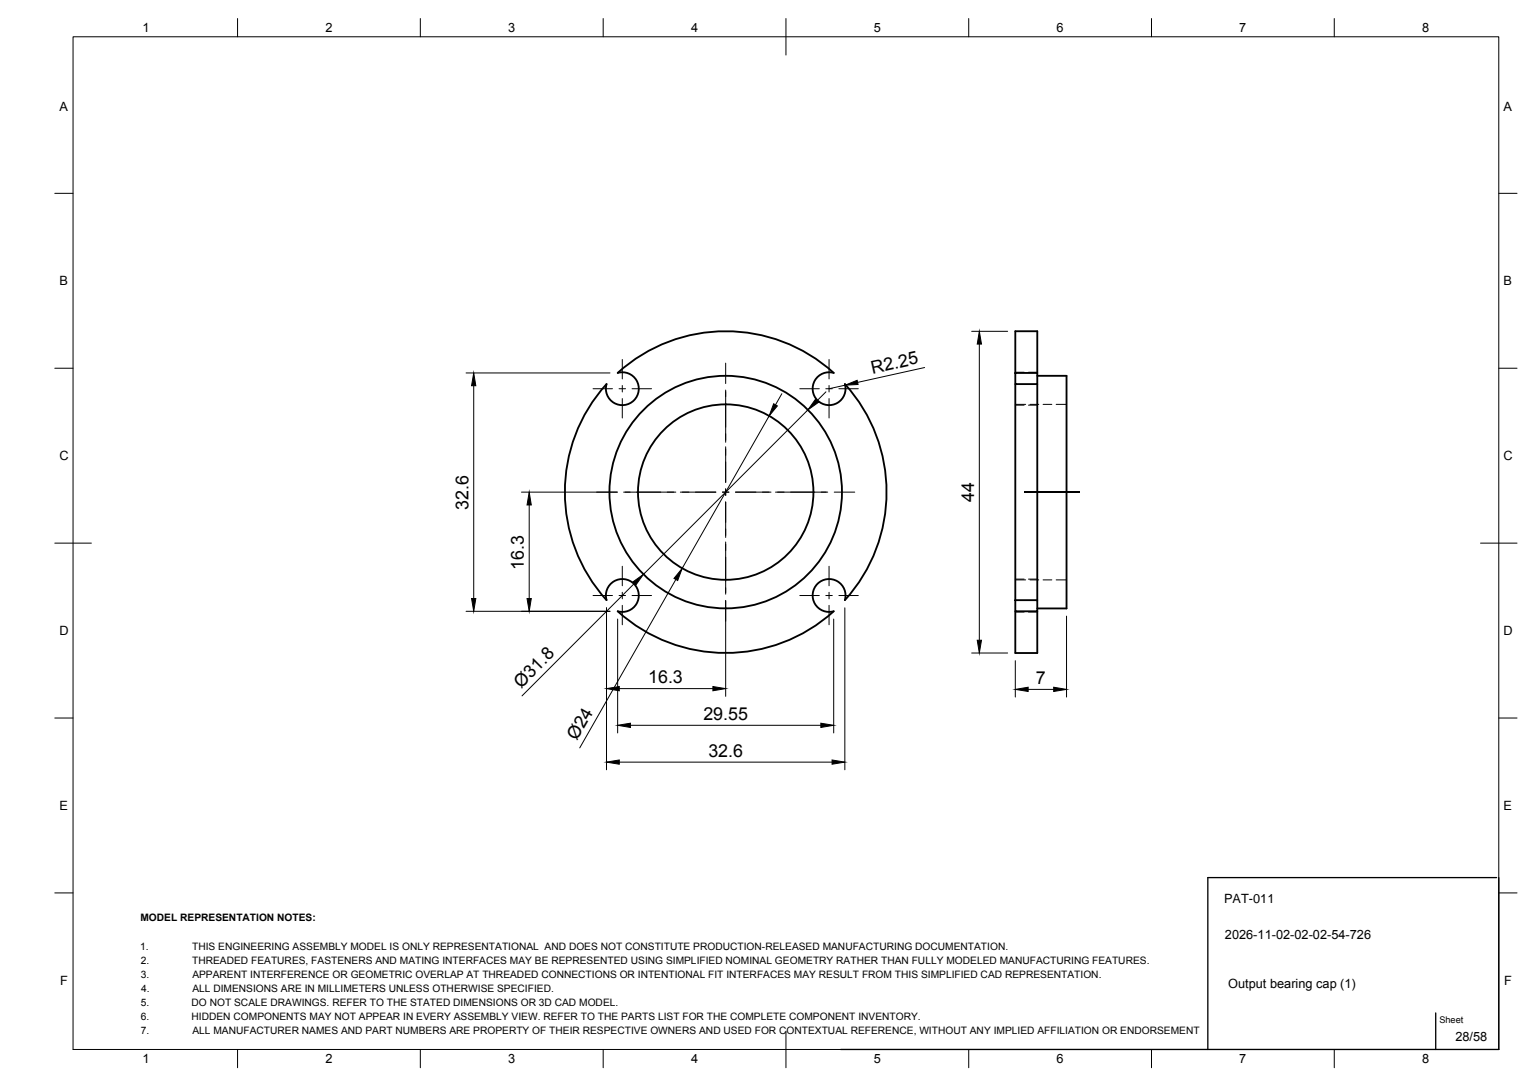
ISO-10303-21;
HEADER;
/* Generated by software containing ST-Developer
 * from STEP Tools, Inc. (www.steptools.com) 
 */

FILE_DESCRIPTION(
/* description */ ('Belt tension measurement rig'),
/* implementation_level */ '2;1');

FILE_NAME(
/* name */ 'Output bearing cap (1).step',
/* time_stamp */ '2026-10-28T03:24:44-07:00',
/* author */ (''),
/* organization */ (''),
/* preprocessor_version */ 'ST-DEVELOPER v20.2',
/* originating_system */ 'Autodesk Translation Framework v15.17.0.0',
/* authorisation */ '');

FILE_SCHEMA (('AUTOMOTIVE_DESIGN { 1 0 10303 214 3 1 1 }'));
ENDSEC;

DATA;
#10=MECHANICAL_DESIGN_GEOMETRIC_PRESENTATION_REPRESENTATION('',(#723),#23587);
#605=SHAPE_REPRESENTATION_RELATIONSHIP('SRR','None',#23852,#660);
#660=ADVANCED_BREP_SHAPE_REPRESENTATION('',(#793),#23550);
#723=STYLED_ITEM('',(#24211),#793);
#793=MANIFOLD_SOLID_BREP('Body1',#12228);
#959=FACE_BOUND('',#2479,.T.);
#960=FACE_BOUND('',#2486,.T.);
#961=FACE_BOUND('',#2489,.T.);
#1180=PLANE('',#13503);
#1181=PLANE('',#13519);
#1182=PLANE('',#13523);
#1640=FACE_OUTER_BOUND('',#2474,.T.);
#1641=FACE_OUTER_BOUND('',#2475,.T.);
#1642=FACE_OUTER_BOUND('',#2476,.T.);
#1643=FACE_OUTER_BOUND('',#2477,.T.);
#1644=FACE_OUTER_BOUND('',#2478,.T.);
#1645=FACE_OUTER_BOUND('',#2480,.T.);
#1646=FACE_OUTER_BOUND('',#2481,.T.);
#1647=FACE_OUTER_BOUND('',#2482,.T.);
#1648=FACE_OUTER_BOUND('',#2483,.T.);
#1649=FACE_OUTER_BOUND('',#2484,.T.);
#1650=FACE_OUTER_BOUND('',#2485,.T.);
#1651=FACE_OUTER_BOUND('',#2487,.T.);
#1652=FACE_OUTER_BOUND('',#2488,.T.);
#2474=EDGE_LOOP('',(#9202,#9203,#9204,#9205));
#2475=EDGE_LOOP('',(#9206,#9207,#9208,#9209));
#2476=EDGE_LOOP('',(#9210,#9211,#9212,#9213));
#2477=EDGE_LOOP('',(#9214,#9215,#9216,#9217));
#2478=EDGE_LOOP('',(#9218,#9219,#9220,#9221,#9222,#9223,#9224,#9225));
#2479=EDGE_LOOP('',(#9226));
#2480=EDGE_LOOP('',(#9227,#9228,#9229,#9230));
#2481=EDGE_LOOP('',(#9231,#9232,#9233,#9234));
#2482=EDGE_LOOP('',(#9235,#9236,#9237,#9238));
#2483=EDGE_LOOP('',(#9239,#9240,#9241,#9242));
#2484=EDGE_LOOP('',(#9243,#9244,#9245,#9246));
#2485=EDGE_LOOP('',(#9247));
#2486=EDGE_LOOP('',(#9248));
#2487=EDGE_LOOP('',(#9249,#9250,#9251,#9252));
#2488=EDGE_LOOP('',(#9253,#9254,#9255,#9256,#9257,#9258,#9259,#9260));
#2489=EDGE_LOOP('',(#9261));
#3284=LINE('',#20344,#4035);
#3285=LINE('',#20348,#4036);
#3286=LINE('',#20353,#4037);
#3287=LINE('',#20357,#4038);
#3288=LINE('',#20362,#4039);
#3289=LINE('',#20366,#4040);
#3290=LINE('',#20371,#4041);
#3291=LINE('',#20375,#4042);
#3292=LINE('',#20394,#4043);
#3293=LINE('',#20402,#4044);
#4035=VECTOR('',#16065,1.);
#4036=VECTOR('',#16068,1.);
#4037=VECTOR('',#16073,1.);
#4038=VECTOR('',#16076,1.);
#4039=VECTOR('',#16081,1.);
#4040=VECTOR('',#16084,1.);
#4041=VECTOR('',#16089,1.);
#4042=VECTOR('',#16092,1.);
#4043=VECTOR('',#16125,1.59);
#4044=VECTOR('',#16136,1.2);
#4764=CIRCLE('',#13492,0.225);
#4765=CIRCLE('',#13493,0.225);
#4766=CIRCLE('',#13495,0.225);
#4767=CIRCLE('',#13496,0.225);
#4768=CIRCLE('',#13498,0.225);
#4769=CIRCLE('',#13499,0.225);
#4770=CIRCLE('',#13501,0.225);
#4771=CIRCLE('',#13502,0.225);
#4772=CIRCLE('',#13504,2.2);
#4773=CIRCLE('',#13505,2.2);
#4774=CIRCLE('',#13506,2.2);
#4775=CIRCLE('',#13507,2.2);
#4776=CIRCLE('',#13508,1.59);
#4777=CIRCLE('',#13510,2.2);
#4778=CIRCLE('',#13512,2.2);
#4779=CIRCLE('',#13514,2.2);
#4780=CIRCLE('',#13516,2.2);
#4781=CIRCLE('',#13518,1.59);
#4782=CIRCLE('',#13520,1.2);
#4783=CIRCLE('',#13522,1.2);
#5666=VERTEX_POINT('',#20342);
#5667=VERTEX_POINT('',#20343);
#5668=VERTEX_POINT('',#20345);
#5669=VERTEX_POINT('',#20347);
#5670=VERTEX_POINT('',#20351);
#5671=VERTEX_POINT('',#20352);
#5672=VERTEX_POINT('',#20354);
#5673=VERTEX_POINT('',#20356);
#5674=VERTEX_POINT('',#20360);
#5675=VERTEX_POINT('',#20361);
#5676=VERTEX_POINT('',#20363);
#5677=VERTEX_POINT('',#20365);
#5678=VERTEX_POINT('',#20369);
#5679=VERTEX_POINT('',#20370);
#5680=VERTEX_POINT('',#20372);
#5681=VERTEX_POINT('',#20374);
#5682=VERTEX_POINT('',#20382);
#5683=VERTEX_POINT('',#20393);
#5684=VERTEX_POINT('',#20397);
#5685=VERTEX_POINT('',#20400);
#6960=EDGE_CURVE('',#5666,#5667,#3284,.T.);
#6961=EDGE_CURVE('',#5668,#5666,#4764,.T.);
#6962=EDGE_CURVE('',#5669,#5668,#3285,.T.);
#6963=EDGE_CURVE('',#5667,#5669,#4765,.T.);
#6964=EDGE_CURVE('',#5670,#5671,#3286,.T.);
#6965=EDGE_CURVE('',#5672,#5670,#4766,.T.);
#6966=EDGE_CURVE('',#5673,#5672,#3287,.T.);
#6967=EDGE_CURVE('',#5671,#5673,#4767,.T.);
#6968=EDGE_CURVE('',#5674,#5675,#3288,.T.);
#6969=EDGE_CURVE('',#5676,#5674,#4768,.T.);
#6970=EDGE_CURVE('',#5677,#5676,#3289,.T.);
#6971=EDGE_CURVE('',#5675,#5677,#4769,.T.);
#6972=EDGE_CURVE('',#5678,#5679,#3290,.T.);
#6973=EDGE_CURVE('',#5680,#5678,#4770,.T.);
#6974=EDGE_CURVE('',#5681,#5680,#3291,.T.);
#6975=EDGE_CURVE('',#5679,#5681,#4771,.T.);
#6976=EDGE_CURVE('',#5680,#5666,#4772,.T.);
#6977=EDGE_CURVE('',#5676,#5678,#4773,.T.);
#6978=EDGE_CURVE('',#5672,#5674,#4774,.T.);
#6979=EDGE_CURVE('',#5668,#5670,#4775,.T.);
#6980=EDGE_CURVE('',#5682,#5682,#4776,.T.);
#6981=EDGE_CURVE('',#5677,#5679,#4777,.T.);
#6982=EDGE_CURVE('',#5673,#5675,#4778,.T.);
#6983=EDGE_CURVE('',#5681,#5667,#4779,.T.);
#6984=EDGE_CURVE('',#5669,#5671,#4780,.T.);
#6985=EDGE_CURVE('',#5682,#5683,#3292,.T.);
#6986=EDGE_CURVE('',#5683,#5683,#4781,.T.);
#6987=EDGE_CURVE('',#5684,#5684,#4782,.T.);
#6988=EDGE_CURVE('',#5685,#5685,#4783,.T.);
#6989=EDGE_CURVE('',#5685,#5684,#3293,.T.);
#9202=ORIENTED_EDGE('',*,*,#6960,.F.);
#9203=ORIENTED_EDGE('',*,*,#6961,.F.);
#9204=ORIENTED_EDGE('',*,*,#6962,.F.);
#9205=ORIENTED_EDGE('',*,*,#6963,.F.);
#9206=ORIENTED_EDGE('',*,*,#6964,.F.);
#9207=ORIENTED_EDGE('',*,*,#6965,.F.);
#9208=ORIENTED_EDGE('',*,*,#6966,.F.);
#9209=ORIENTED_EDGE('',*,*,#6967,.F.);
#9210=ORIENTED_EDGE('',*,*,#6968,.F.);
#9211=ORIENTED_EDGE('',*,*,#6969,.F.);
#9212=ORIENTED_EDGE('',*,*,#6970,.F.);
#9213=ORIENTED_EDGE('',*,*,#6971,.F.);
#9214=ORIENTED_EDGE('',*,*,#6972,.F.);
#9215=ORIENTED_EDGE('',*,*,#6973,.F.);
#9216=ORIENTED_EDGE('',*,*,#6974,.F.);
#9217=ORIENTED_EDGE('',*,*,#6975,.F.);
#9218=ORIENTED_EDGE('',*,*,#6961,.T.);
#9219=ORIENTED_EDGE('',*,*,#6976,.F.);
#9220=ORIENTED_EDGE('',*,*,#6973,.T.);
#9221=ORIENTED_EDGE('',*,*,#6977,.F.);
#9222=ORIENTED_EDGE('',*,*,#6969,.T.);
#9223=ORIENTED_EDGE('',*,*,#6978,.F.);
#9224=ORIENTED_EDGE('',*,*,#6965,.T.);
#9225=ORIENTED_EDGE('',*,*,#6979,.F.);
#9226=ORIENTED_EDGE('',*,*,#6980,.T.);
#9227=ORIENTED_EDGE('',*,*,#6970,.T.);
#9228=ORIENTED_EDGE('',*,*,#6977,.T.);
#9229=ORIENTED_EDGE('',*,*,#6972,.T.);
#9230=ORIENTED_EDGE('',*,*,#6981,.F.);
#9231=ORIENTED_EDGE('',*,*,#6966,.T.);
#9232=ORIENTED_EDGE('',*,*,#6978,.T.);
#9233=ORIENTED_EDGE('',*,*,#6968,.T.);
#9234=ORIENTED_EDGE('',*,*,#6982,.F.);
#9235=ORIENTED_EDGE('',*,*,#6960,.T.);
#9236=ORIENTED_EDGE('',*,*,#6983,.F.);
#9237=ORIENTED_EDGE('',*,*,#6974,.T.);
#9238=ORIENTED_EDGE('',*,*,#6976,.T.);
#9239=ORIENTED_EDGE('',*,*,#6962,.T.);
#9240=ORIENTED_EDGE('',*,*,#6979,.T.);
#9241=ORIENTED_EDGE('',*,*,#6964,.T.);
#9242=ORIENTED_EDGE('',*,*,#6984,.F.);
#9243=ORIENTED_EDGE('',*,*,#6980,.F.);
#9244=ORIENTED_EDGE('',*,*,#6985,.T.);
#9245=ORIENTED_EDGE('',*,*,#6986,.T.);
#9246=ORIENTED_EDGE('',*,*,#6985,.F.);
#9247=ORIENTED_EDGE('',*,*,#6986,.F.);
#9248=ORIENTED_EDGE('',*,*,#6987,.F.);
#9249=ORIENTED_EDGE('',*,*,#6988,.F.);
#9250=ORIENTED_EDGE('',*,*,#6989,.T.);
#9251=ORIENTED_EDGE('',*,*,#6987,.T.);
#9252=ORIENTED_EDGE('',*,*,#6989,.F.);
#9253=ORIENTED_EDGE('',*,*,#6963,.T.);
#9254=ORIENTED_EDGE('',*,*,#6984,.T.);
#9255=ORIENTED_EDGE('',*,*,#6967,.T.);
#9256=ORIENTED_EDGE('',*,*,#6982,.T.);
#9257=ORIENTED_EDGE('',*,*,#6971,.T.);
#9258=ORIENTED_EDGE('',*,*,#6981,.T.);
#9259=ORIENTED_EDGE('',*,*,#6975,.T.);
#9260=ORIENTED_EDGE('',*,*,#6983,.T.);
#9261=ORIENTED_EDGE('',*,*,#6988,.T.);
#11281=CYLINDRICAL_SURFACE('',#13491,0.225);
#11282=CYLINDRICAL_SURFACE('',#13494,0.225);
#11283=CYLINDRICAL_SURFACE('',#13497,0.225);
#11284=CYLINDRICAL_SURFACE('',#13500,0.225);
#11285=CYLINDRICAL_SURFACE('',#13509,2.2);
#11286=CYLINDRICAL_SURFACE('',#13511,2.2);
#11287=CYLINDRICAL_SURFACE('',#13513,2.2);
#11288=CYLINDRICAL_SURFACE('',#13515,2.2);
#11289=CYLINDRICAL_SURFACE('',#13517,1.59);
#11290=CYLINDRICAL_SURFACE('',#13521,1.2);
#11781=ADVANCED_FACE('',(#1640),#11281,.F.);
#11782=ADVANCED_FACE('',(#1641),#11282,.F.);
#11783=ADVANCED_FACE('',(#1642),#11283,.F.);
#11784=ADVANCED_FACE('',(#1643),#11284,.F.);
#11785=ADVANCED_FACE('',(#1644,#959),#1180,.F.);
#11786=ADVANCED_FACE('',(#1645),#11285,.T.);
#11787=ADVANCED_FACE('',(#1646),#11286,.T.);
#11788=ADVANCED_FACE('',(#1647),#11287,.T.);
#11789=ADVANCED_FACE('',(#1648),#11288,.T.);
#11790=ADVANCED_FACE('',(#1649),#11289,.T.);
#11791=ADVANCED_FACE('',(#1650,#960),#1181,.F.);
#11792=ADVANCED_FACE('',(#1651),#11290,.F.);
#11793=ADVANCED_FACE('',(#1652,#961),#1182,.T.);
#12228=CLOSED_SHELL('',(#11781,#11782,#11783,#11784,#11785,#11786,#11787,
#11788,#11789,#11790,#11791,#11792,#11793));
#13490=AXIS2_PLACEMENT_3D('',#20340,#16061,#16062);
#13491=AXIS2_PLACEMENT_3D('',#20341,#16063,#16064);
#13492=AXIS2_PLACEMENT_3D('',#20346,#16066,#16067);
#13493=AXIS2_PLACEMENT_3D('',#20349,#16069,#16070);
#13494=AXIS2_PLACEMENT_3D('',#20350,#16071,#16072);
#13495=AXIS2_PLACEMENT_3D('',#20355,#16074,#16075);
#13496=AXIS2_PLACEMENT_3D('',#20358,#16077,#16078);
#13497=AXIS2_PLACEMENT_3D('',#20359,#16079,#16080);
#13498=AXIS2_PLACEMENT_3D('',#20364,#16082,#16083);
#13499=AXIS2_PLACEMENT_3D('',#20367,#16085,#16086);
#13500=AXIS2_PLACEMENT_3D('',#20368,#16087,#16088);
#13501=AXIS2_PLACEMENT_3D('',#20373,#16090,#16091);
#13502=AXIS2_PLACEMENT_3D('',#20376,#16093,#16094);
#13503=AXIS2_PLACEMENT_3D('',#20377,#16095,#16096);
#13504=AXIS2_PLACEMENT_3D('',#20378,#16097,#16098);
#13505=AXIS2_PLACEMENT_3D('',#20379,#16099,#16100);
#13506=AXIS2_PLACEMENT_3D('',#20380,#16101,#16102);
#13507=AXIS2_PLACEMENT_3D('',#20381,#16103,#16104);
#13508=AXIS2_PLACEMENT_3D('',#20383,#16105,#16106);
#13509=AXIS2_PLACEMENT_3D('',#20384,#16107,#16108);
#13510=AXIS2_PLACEMENT_3D('',#20385,#16109,#16110);
#13511=AXIS2_PLACEMENT_3D('',#20386,#16111,#16112);
#13512=AXIS2_PLACEMENT_3D('',#20387,#16113,#16114);
#13513=AXIS2_PLACEMENT_3D('',#20388,#16115,#16116);
#13514=AXIS2_PLACEMENT_3D('',#20389,#16117,#16118);
#13515=AXIS2_PLACEMENT_3D('',#20390,#16119,#16120);
#13516=AXIS2_PLACEMENT_3D('',#20391,#16121,#16122);
#13517=AXIS2_PLACEMENT_3D('',#20392,#16123,#16124);
#13518=AXIS2_PLACEMENT_3D('',#20395,#16126,#16127);
#13519=AXIS2_PLACEMENT_3D('',#20396,#16128,#16129);
#13520=AXIS2_PLACEMENT_3D('',#20398,#16130,#16131);
#13521=AXIS2_PLACEMENT_3D('',#20399,#16132,#16133);
#13522=AXIS2_PLACEMENT_3D('',#20401,#16134,#16135);
#13523=AXIS2_PLACEMENT_3D('',#20403,#16137,#16138);
#16061=DIRECTION('axis',(0.,0.,1.));
#16062=DIRECTION('refdir',(1.,0.,0.));
#16063=DIRECTION('center_axis',(0.,1.,0.));
#16064=DIRECTION('ref_axis',(0.707106781186549,0.,0.707106781186546));
#16065=DIRECTION('',(0.,1.,0.));
#16066=DIRECTION('center_axis',(0.,1.,0.));
#16067=DIRECTION('ref_axis',(1.,0.,0.));
#16068=DIRECTION('',(0.,-1.,0.));
#16069=DIRECTION('center_axis',(0.,-1.,0.));
#16070=DIRECTION('ref_axis',(1.,0.,0.));
#16071=DIRECTION('center_axis',(0.,1.,0.));
#16072=DIRECTION('ref_axis',(0.707106781186547,0.,-0.707106781186548));
#16073=DIRECTION('',(0.,1.,0.));
#16074=DIRECTION('center_axis',(0.,1.,0.));
#16075=DIRECTION('ref_axis',(1.,0.,0.));
#16076=DIRECTION('',(0.,-1.,0.));
#16077=DIRECTION('center_axis',(0.,-1.,0.));
#16078=DIRECTION('ref_axis',(1.,0.,0.));
#16079=DIRECTION('center_axis',(0.,1.,0.));
#16080=DIRECTION('ref_axis',(-0.707106781186548,0.,-0.707106781186547));
#16081=DIRECTION('',(0.,1.,0.));
#16082=DIRECTION('center_axis',(0.,1.,0.));
#16083=DIRECTION('ref_axis',(1.,0.,0.));
#16084=DIRECTION('',(0.,-1.,0.));
#16085=DIRECTION('center_axis',(0.,-1.,0.));
#16086=DIRECTION('ref_axis',(1.,0.,0.));
#16087=DIRECTION('center_axis',(0.,1.,0.));
#16088=DIRECTION('ref_axis',(-0.707106781186552,0.,0.707106781186543));
#16089=DIRECTION('',(0.,1.,0.));
#16090=DIRECTION('center_axis',(0.,1.,0.));
#16091=DIRECTION('ref_axis',(1.,0.,0.));
#16092=DIRECTION('',(0.,-1.,0.));
#16093=DIRECTION('center_axis',(0.,-1.,0.));
#16094=DIRECTION('ref_axis',(1.,0.,0.));
#16095=DIRECTION('center_axis',(0.,1.,0.));
#16096=DIRECTION('ref_axis',(1.,0.,0.));
#16097=DIRECTION('center_axis',(0.,1.,0.));
#16098=DIRECTION('ref_axis',(1.,0.,0.));
#16099=DIRECTION('center_axis',(0.,1.,0.));
#16100=DIRECTION('ref_axis',(1.,0.,0.));
#16101=DIRECTION('center_axis',(0.,1.,0.));
#16102=DIRECTION('ref_axis',(1.,0.,0.));
#16103=DIRECTION('center_axis',(0.,1.,0.));
#16104=DIRECTION('ref_axis',(1.,0.,0.));
#16105=DIRECTION('center_axis',(0.,1.,0.));
#16106=DIRECTION('ref_axis',(1.,0.,0.));
#16107=DIRECTION('center_axis',(0.,1.,0.));
#16108=DIRECTION('ref_axis',(1.,0.,0.));
#16109=DIRECTION('center_axis',(0.,1.,0.));
#16110=DIRECTION('ref_axis',(1.,0.,0.));
#16111=DIRECTION('center_axis',(0.,1.,0.));
#16112=DIRECTION('ref_axis',(1.,0.,0.));
#16113=DIRECTION('center_axis',(0.,1.,0.));
#16114=DIRECTION('ref_axis',(1.,0.,0.));
#16115=DIRECTION('center_axis',(0.,1.,0.));
#16116=DIRECTION('ref_axis',(1.,0.,0.));
#16117=DIRECTION('center_axis',(0.,1.,0.));
#16118=DIRECTION('ref_axis',(1.,0.,0.));
#16119=DIRECTION('center_axis',(0.,1.,0.));
#16120=DIRECTION('ref_axis',(-1.,0.,-1.22464679914735E-16));
#16121=DIRECTION('center_axis',(0.,1.,0.));
#16122=DIRECTION('ref_axis',(1.,0.,0.));
#16123=DIRECTION('center_axis',(0.,1.,0.));
#16124=DIRECTION('ref_axis',(1.,0.,0.));
#16125=DIRECTION('',(0.,-1.,0.));
#16126=DIRECTION('center_axis',(0.,1.,0.));
#16127=DIRECTION('ref_axis',(1.,0.,0.));
#16128=DIRECTION('center_axis',(0.,1.,0.));
#16129=DIRECTION('ref_axis',(1.,0.,0.));
#16130=DIRECTION('center_axis',(0.,-1.,0.));
#16131=DIRECTION('ref_axis',(1.,0.,0.));
#16132=DIRECTION('center_axis',(0.,1.,0.));
#16133=DIRECTION('ref_axis',(1.,0.,0.));
#16134=DIRECTION('center_axis',(0.,-1.,0.));
#16135=DIRECTION('ref_axis',(1.,0.,0.));
#16136=DIRECTION('',(0.,-1.,0.));
#16137=DIRECTION('center_axis',(0.,1.,0.));
#16138=DIRECTION('ref_axis',(1.,0.,0.));
#20340=CARTESIAN_POINT('',(0.,0.,0.));
#20341=CARTESIAN_POINT('Origin',(8.5857864376269,1.7,5.58578643762691));
#20342=CARTESIAN_POINT('',(8.52266468006184,1.8,5.3698219874924));
#20343=CARTESIAN_POINT('',(8.52266468006184,2.1,5.3698219874924));
#20344=CARTESIAN_POINT('',(8.52266468006184,1.7,5.3698219874924));
#20345=CARTESIAN_POINT('',(8.3698219874924,1.8,5.52266468006184));
#20346=CARTESIAN_POINT('Origin',(8.5857864376269,1.8,5.58578643762691));
#20347=CARTESIAN_POINT('',(8.3698219874924,2.1,5.52266468006184));
#20348=CARTESIAN_POINT('',(8.3698219874924,1.7,5.52266468006184));
#20349=CARTESIAN_POINT('Origin',(8.5857864376269,2.1,5.58578643762691));
#20350=CARTESIAN_POINT('Origin',(8.5857864376269,1.7,8.4142135623731));
#20351=CARTESIAN_POINT('',(8.3698219874924,1.8,8.47733531993816));
#20352=CARTESIAN_POINT('',(8.3698219874924,2.1,8.47733531993816));
#20353=CARTESIAN_POINT('',(8.3698219874924,1.7,8.47733531993816));
#20354=CARTESIAN_POINT('',(8.52266468006184,1.8,8.6301780125076));
#20355=CARTESIAN_POINT('Origin',(8.5857864376269,1.8,8.4142135623731));
#20356=CARTESIAN_POINT('',(8.52266468006184,2.1,8.6301780125076));
#20357=CARTESIAN_POINT('',(8.52266468006184,1.7,8.6301780125076));
#20358=CARTESIAN_POINT('Origin',(8.5857864376269,2.1,8.4142135623731));
#20359=CARTESIAN_POINT('Origin',(11.4142135623731,1.7,8.4142135623731));
#20360=CARTESIAN_POINT('',(11.4773353199382,1.8,8.6301780125076));
#20361=CARTESIAN_POINT('',(11.4773353199382,2.1,8.6301780125076));
#20362=CARTESIAN_POINT('',(11.4773353199382,1.7,8.6301780125076));
#20363=CARTESIAN_POINT('',(11.6301780125076,1.8,8.47733531993816));
#20364=CARTESIAN_POINT('Origin',(11.4142135623731,1.8,8.4142135623731));
#20365=CARTESIAN_POINT('',(11.6301780125076,2.1,8.47733531993816));
#20366=CARTESIAN_POINT('',(11.6301780125076,1.7,8.47733531993816));
#20367=CARTESIAN_POINT('Origin',(11.4142135623731,2.1,8.4142135623731));
#20368=CARTESIAN_POINT('Origin',(11.4142135623731,1.7,5.58578643762691));
#20369=CARTESIAN_POINT('',(11.6301780125076,1.8,5.52266468006184));
#20370=CARTESIAN_POINT('',(11.6301780125076,2.1,5.52266468006184));
#20371=CARTESIAN_POINT('',(11.6301780125076,1.7,5.52266468006184));
#20372=CARTESIAN_POINT('',(11.4773353199382,1.8,5.3698219874924));
#20373=CARTESIAN_POINT('Origin',(11.4142135623731,1.8,5.58578643762691));
#20374=CARTESIAN_POINT('',(11.4773353199382,2.1,5.3698219874924));
#20375=CARTESIAN_POINT('',(11.4773353199382,1.7,5.3698219874924));
#20376=CARTESIAN_POINT('Origin',(11.4142135623731,2.1,5.58578643762691));
#20377=CARTESIAN_POINT('Origin',(10.,1.8,7.));
#20378=CARTESIAN_POINT('Origin',(10.,1.8,7.));
#20379=CARTESIAN_POINT('Origin',(10.,1.8,7.));
#20380=CARTESIAN_POINT('Origin',(10.,1.8,7.));
#20381=CARTESIAN_POINT('Origin',(10.,1.8,7.));
#20382=CARTESIAN_POINT('',(8.41,1.8,7.));
#20383=CARTESIAN_POINT('Origin',(10.,1.8,7.));
#20384=CARTESIAN_POINT('Origin',(10.,1.8,7.));
#20385=CARTESIAN_POINT('Origin',(10.,2.1,7.));
#20386=CARTESIAN_POINT('Origin',(10.,1.8,7.));
#20387=CARTESIAN_POINT('Origin',(10.,2.1,7.));
#20388=CARTESIAN_POINT('Origin',(10.,1.8,7.));
#20389=CARTESIAN_POINT('Origin',(10.,2.1,7.));
#20390=CARTESIAN_POINT('Origin',(10.,1.8,7.));
#20391=CARTESIAN_POINT('Origin',(10.,2.1,7.));
#20392=CARTESIAN_POINT('Origin',(10.,1.4,7.));
#20393=CARTESIAN_POINT('',(8.41,1.4,7.));
#20394=CARTESIAN_POINT('',(8.41,1.4,7.));
#20395=CARTESIAN_POINT('Origin',(10.,1.4,7.));
#20396=CARTESIAN_POINT('Origin',(10.,1.4,7.));
#20397=CARTESIAN_POINT('',(8.8,1.4,7.));
#20398=CARTESIAN_POINT('Origin',(10.,1.4,7.));
#20399=CARTESIAN_POINT('Origin',(10.,1.8,7.));
#20400=CARTESIAN_POINT('',(8.8,2.1,7.));
#20401=CARTESIAN_POINT('Origin',(10.,2.1,7.));
#20402=CARTESIAN_POINT('',(8.8,1.8,7.));
#20403=CARTESIAN_POINT('Origin',(10.,2.1,7.));
#23485=UNCERTAINTY_MEASURE_WITH_UNIT(LENGTH_MEASURE(0.001),#23588,
'DISTANCE_ACCURACY_VALUE',
'Maximum model space distance between geometric entities at asserted c
onnectivities');
#23522=UNCERTAINTY_MEASURE_WITH_UNIT(LENGTH_MEASURE(0.001),#23588,
'DISTANCE_ACCURACY_VALUE',
'Maximum model space distance between geometric entities at asserted c
onnectivities');
#23550=(
GEOMETRIC_REPRESENTATION_CONTEXT(3)
GLOBAL_UNCERTAINTY_ASSIGNED_CONTEXT((#23485))
GLOBAL_UNIT_ASSIGNED_CONTEXT((#23588,#23590,#23591))
REPRESENTATION_CONTEXT('','3D')
);
#23587=(
GEOMETRIC_REPRESENTATION_CONTEXT(3)
GLOBAL_UNCERTAINTY_ASSIGNED_CONTEXT((#23522))
GLOBAL_UNIT_ASSIGNED_CONTEXT((#23588,#23590,#23591))
REPRESENTATION_CONTEXT('','3D')
);
#23588=(
LENGTH_UNIT()
NAMED_UNIT(*)
SI_UNIT(.CENTI.,.METRE.)
);
#23590=(
NAMED_UNIT(*)
PLANE_ANGLE_UNIT()
SI_UNIT($,.RADIAN.)
);
#23591=(
NAMED_UNIT(*)
SI_UNIT($,.STERADIAN.)
SOLID_ANGLE_UNIT()
);
#23619=SHAPE_DEFINITION_REPRESENTATION(#23688,#23852);
#23688=PRODUCT_DEFINITION_SHAPE('',$,#23917);
#23852=SHAPE_REPRESENTATION('',(#13490),#23550);
#23889=PRODUCT_DEFINITION_CONTEXT('part definition',#24083,'design');
#23917=PRODUCT_DEFINITION('Output bearing cap (1)',
'Output bearing cap (1)',#23981,#23889);
#23981=PRODUCT_DEFINITION_FORMATION('',$,#24112);
#24083=APPLICATION_CONTEXT(
'Core Data for Automotive Mechanical Design Process');
#24084=PRODUCT_CONTEXT('part definition',#24083,'mechanical');
#24112=PRODUCT('Output bearing cap (1)','Output bearing cap (1)',
'Output bearing cap (1)',(#24084));
#24205=COLOUR_RGB('Grey',0.48,0.52,0.57);
#24206=FILL_AREA_STYLE_COLOUR('',#24205);
#24207=FILL_AREA_STYLE('',(#24206));
#24208=SURFACE_STYLE_FILL_AREA(#24207);
#24209=SURFACE_SIDE_STYLE('',(#24208));
#24210=SURFACE_STYLE_USAGE(.BOTH.,#24209);
#24211=PRESENTATION_STYLE_ASSIGNMENT((#24210));
ENDSEC;
END-ISO-10303-21;
